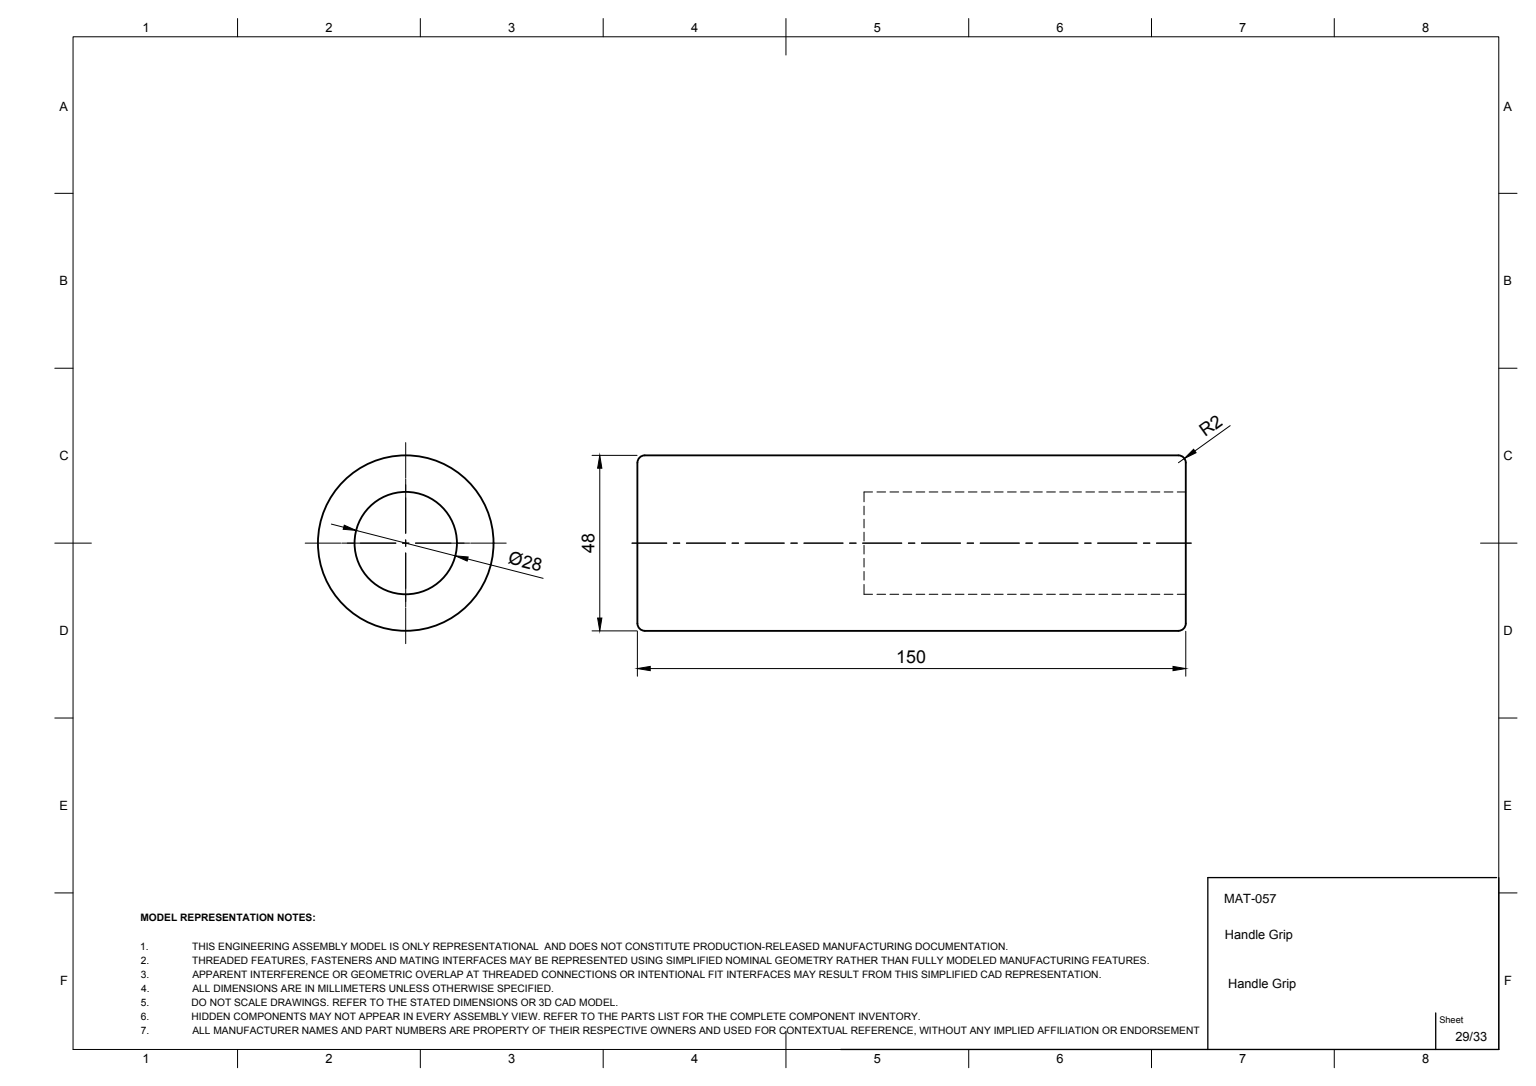
ISO-10303-21;
HEADER;
/* Generated by software containing ST-Developer
 * from STEP Tools, Inc. (www.steptools.com) 
 */

FILE_DESCRIPTION(
/* description */ ('STEP AP214', 'CAx-IF Rec.Pracs.---Representation and Presentation of Product Manufa
cturing Information (PMI)---4.0---2014-10-13'),
/* implementation_level */ '2;1');

FILE_NAME(
/* name */ 'Handle Grip.step',
/* time_stamp */ '2026-10-28T23:34:22+01:00',
/* author */ (''),
/* organization */ (''),
/* preprocessor_version */ 'ST-DEVELOPER v20.2',
/* originating_system */ 'Autodesk Translation Framework v15.17.0.0',
/* authorisation */ '');

FILE_SCHEMA (('AP242_MANAGED_MODEL_BASED_3D_ENGINEERING_MIM_LF { 1 0 10303 442 2 1 4 }'));
ENDSEC;

DATA;
#10=MECHANICAL_DESIGN_GEOMETRIC_PRESENTATION_REPRESENTATION('',(#270),#27807);
#222=SHAPE_REPRESENTATION_RELATIONSHIP('SRR','None',#27920,#244);
#244=ADVANCED_BREP_SHAPE_REPRESENTATION('',(#299),#27800);
#270=STYLED_ITEM('',(#28084),#299);
#299=MANIFOLD_SOLID_BREP('Body1',#12046);
#426=FACE_BOUND('',#2580,.T.);
#690=PLANE('',#13449);
#691=PLANE('',#13450);
#692=PLANE('',#13451);
#840=TOROIDAL_SURFACE('',#13435,22.,2.);
#841=TOROIDAL_SURFACE('',#13440,22.,2.);
#1177=CYLINDRICAL_SURFACE('',#13445,24.);
#1178=CYLINDRICAL_SURFACE('',#13446,14.);
#1786=FACE_OUTER_BOUND('',#2574,.T.);
#1787=FACE_OUTER_BOUND('',#2575,.T.);
#1788=FACE_OUTER_BOUND('',#2576,.T.);
#1789=FACE_OUTER_BOUND('',#2577,.T.);
#1790=FACE_OUTER_BOUND('',#2578,.T.);
#1791=FACE_OUTER_BOUND('',#2579,.T.);
#1792=FACE_OUTER_BOUND('',#2581,.T.);
#2574=EDGE_LOOP('',(#10539,#10540,#10541,#10542,#10543));
#2575=EDGE_LOOP('',(#10544,#10545,#10546,#10547,#10548));
#2576=EDGE_LOOP('',(#10549,#10550,#10551,#10552,#10553,#10554));
#2577=EDGE_LOOP('',(#10555,#10556,#10557,#10558));
#2578=EDGE_LOOP('',(#10559));
#2579=EDGE_LOOP('',(#10560));
#2580=EDGE_LOOP('',(#10561));
#2581=EDGE_LOOP('',(#10562));
#3420=LINE('',#23201,#4240);
#3421=LINE('',#23206,#4241);
#4240=VECTOR('',#16694,24.);
#4241=VECTOR('',#16699,14.);
#4925=CIRCLE('',#13436,22.);
#4926=CIRCLE('',#13437,2.);
#4927=CIRCLE('',#13438,24.);
#4928=CIRCLE('',#13439,24.);
#4929=CIRCLE('',#13441,24.);
#4930=CIRCLE('',#13442,24.);
#4931=CIRCLE('',#13443,2.);
#4932=CIRCLE('',#13444,22.);
#4933=CIRCLE('',#13447,14.);
#4934=CIRCLE('',#13448,14.);
#5897=VERTEX_POINT('',#23185);
#5898=VERTEX_POINT('',#23187);
#5899=VERTEX_POINT('',#23189);
#5900=VERTEX_POINT('',#23193);
#5901=VERTEX_POINT('',#23194);
#5902=VERTEX_POINT('',#23197);
#5903=VERTEX_POINT('',#23203);
#5904=VERTEX_POINT('',#23205);
#7482=EDGE_CURVE('',#5897,#5897,#4925,.T.);
#7483=EDGE_CURVE('',#5897,#5898,#4926,.T.);
#7484=EDGE_CURVE('',#5899,#5898,#4927,.T.);
#7485=EDGE_CURVE('',#5898,#5899,#4928,.T.);
#7486=EDGE_CURVE('',#5900,#5901,#4929,.T.);
#7487=EDGE_CURVE('',#5901,#5900,#4930,.T.);
#7488=EDGE_CURVE('',#5901,#5902,#4931,.T.);
#7489=EDGE_CURVE('',#5902,#5902,#4932,.T.);
#7490=EDGE_CURVE('',#5900,#5899,#3420,.T.);
#7491=EDGE_CURVE('',#5903,#5903,#4933,.T.);
#7492=EDGE_CURVE('',#5903,#5904,#3421,.T.);
#7493=EDGE_CURVE('',#5904,#5904,#4934,.T.);
#10539=ORIENTED_EDGE('',*,*,#7482,.F.);
#10540=ORIENTED_EDGE('',*,*,#7483,.T.);
#10541=ORIENTED_EDGE('',*,*,#7484,.F.);
#10542=ORIENTED_EDGE('',*,*,#7485,.F.);
#10543=ORIENTED_EDGE('',*,*,#7483,.F.);
#10544=ORIENTED_EDGE('',*,*,#7486,.F.);
#10545=ORIENTED_EDGE('',*,*,#7487,.F.);
#10546=ORIENTED_EDGE('',*,*,#7488,.T.);
#10547=ORIENTED_EDGE('',*,*,#7489,.F.);
#10548=ORIENTED_EDGE('',*,*,#7488,.F.);
#10549=ORIENTED_EDGE('',*,*,#7486,.T.);
#10550=ORIENTED_EDGE('',*,*,#7487,.T.);
#10551=ORIENTED_EDGE('',*,*,#7490,.T.);
#10552=ORIENTED_EDGE('',*,*,#7484,.T.);
#10553=ORIENTED_EDGE('',*,*,#7485,.T.);
#10554=ORIENTED_EDGE('',*,*,#7490,.F.);
#10555=ORIENTED_EDGE('',*,*,#7491,.T.);
#10556=ORIENTED_EDGE('',*,*,#7492,.T.);
#10557=ORIENTED_EDGE('',*,*,#7493,.F.);
#10558=ORIENTED_EDGE('',*,*,#7492,.F.);
#10559=ORIENTED_EDGE('',*,*,#7482,.T.);
#10560=ORIENTED_EDGE('',*,*,#7489,.T.);
#10561=ORIENTED_EDGE('',*,*,#7493,.T.);
#10562=ORIENTED_EDGE('',*,*,#7491,.F.);
#11868=ADVANCED_FACE('',(#1786),#840,.T.);
#11869=ADVANCED_FACE('',(#1787),#841,.T.);
#11870=ADVANCED_FACE('',(#1788),#1177,.T.);
#11871=ADVANCED_FACE('',(#1789),#1178,.F.);
#11872=ADVANCED_FACE('',(#1790),#690,.T.);
#11873=ADVANCED_FACE('',(#1791,#426),#691,.F.);
#11874=ADVANCED_FACE('',(#1792),#692,.F.);
#12046=CLOSED_SHELL('',(#11868,#11869,#11870,#11871,#11872,#11873,#11874));
#13434=AXIS2_PLACEMENT_3D('',#23183,#16670,#16671);
#13435=AXIS2_PLACEMENT_3D('',#23184,#16672,#16673);
#13436=AXIS2_PLACEMENT_3D('',#23186,#16674,#16675);
#13437=AXIS2_PLACEMENT_3D('',#23188,#16676,#16677);
#13438=AXIS2_PLACEMENT_3D('',#23190,#16678,#16679);
#13439=AXIS2_PLACEMENT_3D('',#23191,#16680,#16681);
#13440=AXIS2_PLACEMENT_3D('',#23192,#16682,#16683);
#13441=AXIS2_PLACEMENT_3D('',#23195,#16684,#16685);
#13442=AXIS2_PLACEMENT_3D('',#23196,#16686,#16687);
#13443=AXIS2_PLACEMENT_3D('',#23198,#16688,#16689);
#13444=AXIS2_PLACEMENT_3D('',#23199,#16690,#16691);
#13445=AXIS2_PLACEMENT_3D('',#23200,#16692,#16693);
#13446=AXIS2_PLACEMENT_3D('',#23202,#16695,#16696);
#13447=AXIS2_PLACEMENT_3D('',#23204,#16697,#16698);
#13448=AXIS2_PLACEMENT_3D('',#23207,#16700,#16701);
#13449=AXIS2_PLACEMENT_3D('',#23208,#16702,#16703);
#13450=AXIS2_PLACEMENT_3D('',#23209,#16704,#16705);
#13451=AXIS2_PLACEMENT_3D('',#23210,#16706,#16707);
#16670=DIRECTION('axis',(0.,0.,1.));
#16671=DIRECTION('refdir',(1.,0.,0.));
#16672=DIRECTION('center_axis',(0.852431871234063,0.522838316216777,2.44136686633116E-17));
#16673=DIRECTION('ref_axis',(0.522838316216777,-0.852431871234062,0.));
#16674=DIRECTION('center_axis',(0.852431871234063,0.522838316216777,2.44136686633116E-17));
#16675=DIRECTION('ref_axis',(0.522838316216777,-0.852431871234063,1.84889274661175E-32));
#16676=DIRECTION('center_axis',(-2.08109892623551E-17,-1.27644014166001E-17,
1.));
#16677=DIRECTION('ref_axis',(-0.522838316216778,0.852431871234062,0.));
#16678=DIRECTION('center_axis',(-0.852431871234063,-0.522838316216777,-2.44136686633116E-17));
#16679=DIRECTION('ref_axis',(0.522838316216777,-0.852431871234063,-1.54074395550979E-32));
#16680=DIRECTION('center_axis',(-0.852431871234063,-0.522838316216777,-2.44136686633116E-17));
#16681=DIRECTION('ref_axis',(0.522838316216777,-0.852431871234063,-1.54074395550979E-32));
#16682=DIRECTION('center_axis',(0.852431871234063,0.522838316216777,2.44136686633116E-17));
#16683=DIRECTION('ref_axis',(0.522838316216777,-0.852431871234062,0.));
#16684=DIRECTION('center_axis',(0.852431871234063,0.522838316216777,2.44136686633116E-17));
#16685=DIRECTION('ref_axis',(0.522838316216777,-0.852431871234063,-1.54074395550979E-32));
#16686=DIRECTION('center_axis',(0.852431871234063,0.522838316216777,2.44136686633116E-17));
#16687=DIRECTION('ref_axis',(0.522838316216777,-0.852431871234063,-1.54074395550979E-32));
#16688=DIRECTION('center_axis',(-2.08109892623551E-17,-1.27644014166001E-17,
1.));
#16689=DIRECTION('ref_axis',(-0.522838316216776,0.852431871234063,0.));
#16690=DIRECTION('center_axis',(-0.852431871234063,-0.522838316216777,-2.44136686633116E-17));
#16691=DIRECTION('ref_axis',(0.522838316216777,-0.852431871234063,1.84889274661175E-32));
#16692=DIRECTION('center_axis',(-0.852431871234063,-0.522838316216777,-2.44136686633116E-17));
#16693=DIRECTION('ref_axis',(-0.522838316216777,0.852431871234063,1.54074395550979E-32));
#16694=DIRECTION('',(0.852431871234063,0.522838316216777,2.44136686633116E-17));
#16695=DIRECTION('center_axis',(-0.852431871234063,-0.522838316216777,-2.44136686633116E-17));
#16696=DIRECTION('ref_axis',(-0.522838316216777,0.852431871234063,-1.54074395550979E-32));
#16697=DIRECTION('center_axis',(0.852431871234063,0.522838316216777,2.44136686633116E-17));
#16698=DIRECTION('ref_axis',(-0.522838316216777,0.852431871234063,-1.69481835106077E-32));
#16699=DIRECTION('',(-0.852431871234063,-0.522838316216777,-2.44136686633116E-17));
#16700=DIRECTION('center_axis',(0.852431871234063,0.522838316216777,2.44136686633116E-17));
#16701=DIRECTION('ref_axis',(0.522838316216777,-0.852431871234063,1.54074395550979E-32));
#16702=DIRECTION('center_axis',(0.852431871234063,0.522838316216777,2.44136686633116E-17));
#16703=DIRECTION('ref_axis',(0.522838316216777,-0.852431871234063,-1.10549867763274E-16));
#16704=DIRECTION('center_axis',(0.852431871234063,0.522838316216777,2.44136686633116E-17));
#16705=DIRECTION('ref_axis',(0.522838316216777,-0.852431871234063,-1.10549867763274E-16));
#16706=DIRECTION('center_axis',(0.852431871234063,0.522838316216777,2.44136686633116E-17));
#16707=DIRECTION('ref_axis',(-0.522838316216777,0.852431871234063,0.));
#23183=CARTESIAN_POINT('',(0.,0.,0.));
#23184=CARTESIAN_POINT('Origin',(764.341398189025,488.655221713906,260.073593133703));
#23185=CARTESIAN_POINT('',(754.543818974723,508.454399513489,260.073593133703));
#23186=CARTESIAN_POINT('Origin',(766.046261931493,489.70089834634,260.073593133703));
#23187=CARTESIAN_POINT('',(751.793278599822,509.113586623524,260.073593133703));
#23188=CARTESIAN_POINT('Origin',(752.838955232255,507.408722881056,260.073593133703));
#23189=CARTESIAN_POINT('',(776.889517778227,468.196856804289,260.073593133703));
#23190=CARTESIAN_POINT('Origin',(764.341398189025,488.655221713906,260.073593133703));
#23191=CARTESIAN_POINT('Origin',(764.341398189025,488.655221713906,260.073593133703));
#23192=CARTESIAN_POINT('Origin',(639.886344988851,412.320827546257,260.073593133703));
#23193=CARTESIAN_POINT('',(652.434464578054,391.862462636639,260.073593133703));
#23194=CARTESIAN_POINT('',(627.338225399649,432.779192455874,260.073593133703));
#23195=CARTESIAN_POINT('Origin',(639.886344988851,412.320827546257,260.073593133703));
#23196=CARTESIAN_POINT('Origin',(639.886344988851,412.320827546257,260.073593133703));
#23197=CARTESIAN_POINT('',(626.679038289614,430.028652080973,260.073593133703));
#23198=CARTESIAN_POINT('Origin',(628.383902032082,431.074328713406,260.073593133703));
#23199=CARTESIAN_POINT('Origin',(638.181481246383,411.275150913823,260.073593133703));
#23200=CARTESIAN_POINT('Origin',(766.046261931493,489.70089834634,260.073593133703));
#23201=CARTESIAN_POINT('',(778.594381520695,469.242533436722,260.073593133703));
#23202=CARTESIAN_POINT('Origin',(766.046261931493,489.70089834634,260.073593133703));
#23203=CARTESIAN_POINT('',(720.515222342016,445.350876543623,260.073593133703));
#23204=CARTESIAN_POINT('Origin',(713.195485914981,457.2849227409,260.073593133703));
#23205=CARTESIAN_POINT('',(645.501217673418,399.341104716547,260.073593133703));
#23206=CARTESIAN_POINT('',(773.365998358528,477.766852149063,260.073593133703));
#23207=CARTESIAN_POINT('Origin',(638.181481246383,411.275150913823,260.073593133703));
#23208=CARTESIAN_POINT('Origin',(766.046261931493,489.70089834634,260.073593133703));
#23209=CARTESIAN_POINT('Origin',(638.181481246383,411.275150913823,260.073593133703));
#23210=CARTESIAN_POINT('Origin',(713.195485914981,457.2849227409,260.073593133703));
#27771=UNCERTAINTY_MEASURE_WITH_UNIT(LENGTH_MEASURE(0.01),#27808,
'DISTANCE_ACCURACY_VALUE',
'Maximum model space distance between geometric entities at asserted c
onnectivities');
#27778=UNCERTAINTY_MEASURE_WITH_UNIT(LENGTH_MEASURE(0.01),#27808,
'DISTANCE_ACCURACY_VALUE',
'Maximum model space distance between geometric entities at asserted c
onnectivities');
#27800=(
GEOMETRIC_REPRESENTATION_CONTEXT(3)
GLOBAL_UNCERTAINTY_ASSIGNED_CONTEXT((#27771))
GLOBAL_UNIT_ASSIGNED_CONTEXT((#27808,#27810,#27811))
REPRESENTATION_CONTEXT('','3D')
);
#27807=(
GEOMETRIC_REPRESENTATION_CONTEXT(3)
GLOBAL_UNCERTAINTY_ASSIGNED_CONTEXT((#27778))
GLOBAL_UNIT_ASSIGNED_CONTEXT((#27808,#27810,#27811))
REPRESENTATION_CONTEXT('','3D')
);
#27808=(
LENGTH_UNIT()
NAMED_UNIT(*)
SI_UNIT(.MILLI.,.METRE.)
);
#27810=(
NAMED_UNIT(*)
PLANE_ANGLE_UNIT()
SI_UNIT($,.RADIAN.)
);
#27811=(
NAMED_UNIT(*)
SI_UNIT($,.STERADIAN.)
SOLID_ANGLE_UNIT()
);
#27833=SHAPE_DEFINITION_REPRESENTATION(#27873,#27920);
#27873=PRODUCT_DEFINITION_SHAPE('',$,#27949);
#27920=SHAPE_REPRESENTATION('',(#13434),#27800);
#27927=PRODUCT_DEFINITION_CONTEXT('part definition',#28013,'design');
#27949=PRODUCT_DEFINITION('Handle Grip','Handle Grip',#27977,#27927);
#27977=PRODUCT_DEFINITION_FORMATION('',$,#28036);
#28013=APPLICATION_CONTEXT('Managed model based 3d engineering');
#28014=PRODUCT_CONTEXT('part definition',#28013,'mechanical');
#28036=PRODUCT('Handle Grip','Handle Grip',$,(#28014));
#28078=COLOUR_RGB('Black',0.12,0.14,0.17);
#28079=FILL_AREA_STYLE_COLOUR('',#28078);
#28080=FILL_AREA_STYLE('',(#28079));
#28081=SURFACE_STYLE_FILL_AREA(#28080);
#28082=SURFACE_SIDE_STYLE('',(#28081));
#28083=SURFACE_STYLE_USAGE(.BOTH.,#28082);
#28084=PRESENTATION_STYLE_ASSIGNMENT((#28083));
ENDSEC;
END-ISO-10303-21;
